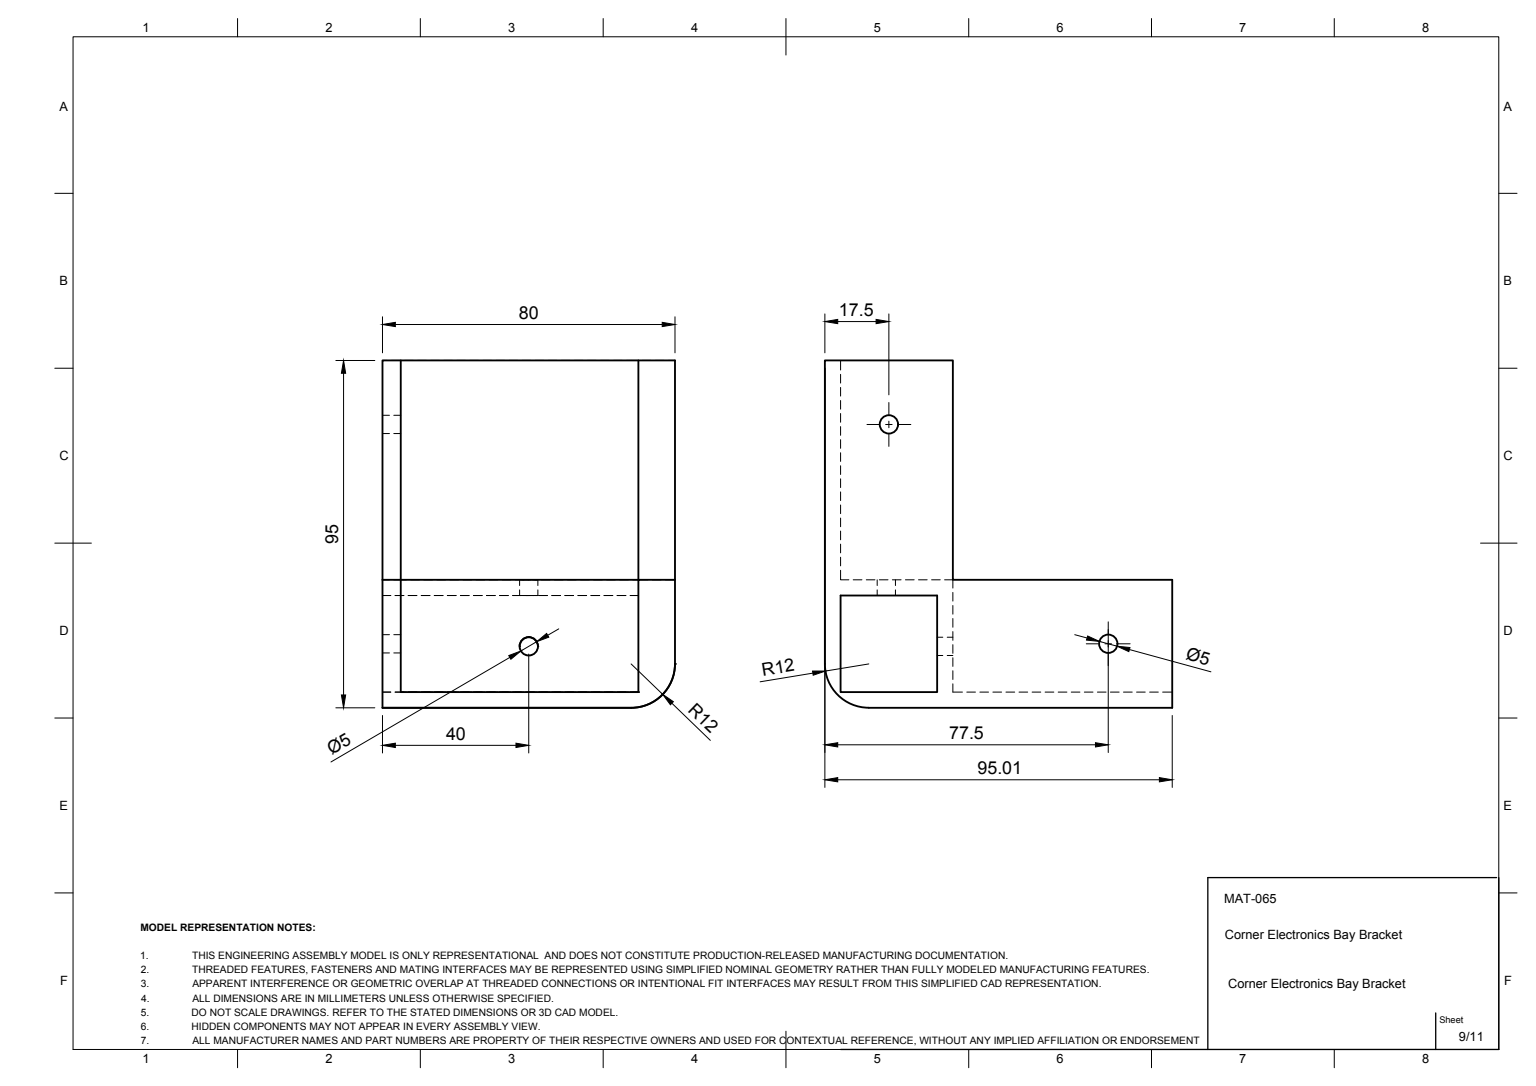
ISO-10303-21;
HEADER;
/* Generated by software containing ST-Developer
 * from STEP Tools, Inc. (www.steptools.com) 
 */

FILE_DESCRIPTION(
/* description */ (
'CAx-IF Rec.Pracs.---Representation and Presentation of Product Manufa
cturing Information (PMI)---4.0---2014-10-13'),
/* implementation_level */ '2;1');

FILE_NAME(
/* name */ 'Corner Electronics Bay Bracket.step',
/* time_stamp */ '2026-11-15T23:28:27-08:00',
/* author */ (''),
/* organization */ (''),
/* preprocessor_version */ 'ST-DEVELOPER v20.2',
/* originating_system */ 'Autodesk Translation Framework v15.17.0.0',
/* authorisation */ '');

FILE_SCHEMA (('AUTOMOTIVE_DESIGN { 1 0 10303 214 3 1 1 }'));
ENDSEC;

DATA;
#10=MECHANICAL_DESIGN_GEOMETRIC_PRESENTATION_REPRESENTATION('',(#196),#7756);
#164=SPHERICAL_SURFACE('',#5002,0.012);
#178=SHAPE_REPRESENTATION_RELATIONSHIP('SRR','None',#7826,#187);
#187=ADVANCED_BREP_SHAPE_REPRESENTATION('',(#205),#7754);
#196=STYLED_ITEM('',(#7874),#205);
#205=MANIFOLD_SOLID_BREP('Body1',#4633);
#239=CYLINDRICAL_SURFACE('',#4970,0.0025);
#240=CYLINDRICAL_SURFACE('',#4977,0.0025);
#241=CYLINDRICAL_SURFACE('',#4988,0.0025);
#242=CYLINDRICAL_SURFACE('',#4989,0.0025);
#243=CYLINDRICAL_SURFACE('',#4996,0.012);
#244=CYLINDRICAL_SURFACE('',#4998,0.012);
#245=CYLINDRICAL_SURFACE('',#5000,0.012);
#328=CIRCLE('',#4959,0.0025);
#329=CIRCLE('',#4963,0.0025);
#330=CIRCLE('',#4967,0.012);
#331=CIRCLE('',#4971,0.0025);
#332=CIRCLE('',#4972,0.0025);
#333=CIRCLE('',#4974,0.0025);
#334=CIRCLE('',#4976,0.012);
#335=CIRCLE('',#4978,0.0025);
#336=CIRCLE('',#4981,0.012);
#337=CIRCLE('',#4983,0.0025);
#338=CIRCLE('',#4987,0.0025);
#339=CIRCLE('',#4997,0.012);
#340=CIRCLE('',#4999,0.012);
#341=CIRCLE('',#5001,0.012);
#420=FACE_BOUND('',#877,.T.);
#421=FACE_BOUND('',#881,.T.);
#422=FACE_BOUND('',#889,.T.);
#423=FACE_BOUND('',#893,.T.);
#424=FACE_BOUND('',#895,.T.);
#425=FACE_BOUND('',#896,.T.);
#426=FACE_BOUND('',#897,.T.);
#427=FACE_BOUND('',#899,.T.);
#428=FACE_BOUND('',#903,.T.);
#601=FACE_OUTER_BOUND('',#876,.T.);
#602=FACE_OUTER_BOUND('',#878,.T.);
#603=FACE_OUTER_BOUND('',#879,.T.);
#604=FACE_OUTER_BOUND('',#880,.T.);
#605=FACE_OUTER_BOUND('',#882,.T.);
#606=FACE_OUTER_BOUND('',#883,.T.);
#607=FACE_OUTER_BOUND('',#884,.T.);
#608=FACE_OUTER_BOUND('',#885,.T.);
#609=FACE_OUTER_BOUND('',#886,.T.);
#610=FACE_OUTER_BOUND('',#887,.T.);
#611=FACE_OUTER_BOUND('',#888,.T.);
#612=FACE_OUTER_BOUND('',#890,.T.);
#613=FACE_OUTER_BOUND('',#891,.T.);
#614=FACE_OUTER_BOUND('',#892,.T.);
#615=FACE_OUTER_BOUND('',#894,.T.);
#616=FACE_OUTER_BOUND('',#898,.T.);
#617=FACE_OUTER_BOUND('',#900,.T.);
#618=FACE_OUTER_BOUND('',#901,.T.);
#619=FACE_OUTER_BOUND('',#902,.T.);
#620=FACE_OUTER_BOUND('',#904,.T.);
#621=FACE_OUTER_BOUND('',#905,.T.);
#622=FACE_OUTER_BOUND('',#906,.T.);
#623=FACE_OUTER_BOUND('',#907,.T.);
#624=FACE_OUTER_BOUND('',#908,.T.);
#625=FACE_OUTER_BOUND('',#909,.T.);
#626=FACE_OUTER_BOUND('',#910,.T.);
#627=FACE_OUTER_BOUND('',#911,.T.);
#628=FACE_OUTER_BOUND('',#912,.T.);
#629=FACE_OUTER_BOUND('',#913,.T.);
#630=FACE_OUTER_BOUND('',#914,.T.);
#631=FACE_OUTER_BOUND('',#915,.T.);
#876=EDGE_LOOP('',(#3789,#3790,#3791,#3792));
#877=EDGE_LOOP('',(#3793));
#878=EDGE_LOOP('',(#3794,#3795,#3796,#3797));
#879=EDGE_LOOP('',(#3798,#3799,#3800,#3801));
#880=EDGE_LOOP('',(#3802,#3803,#3804,#3805));
#881=EDGE_LOOP('',(#3806));
#882=EDGE_LOOP('',(#3807,#3808,#3809,#3810));
#883=EDGE_LOOP('',(#3811,#3812,#3813,#3814));
#884=EDGE_LOOP('',(#3815,#3816,#3817,#3818,#3819,#3820,#3821,#3822,#3823));
#885=EDGE_LOOP('',(#3824,#3825,#3826,#3827));
#886=EDGE_LOOP('',(#3828,#3829,#3830,#3831));
#887=EDGE_LOOP('',(#3832,#3833,#3834,#3835));
#888=EDGE_LOOP('',(#3836,#3837,#3838,#3839));
#889=EDGE_LOOP('',(#3840));
#890=EDGE_LOOP('',(#3841,#3842,#3843,#3844,#3845,#3846,#3847,#3848,#3849));
#891=EDGE_LOOP('',(#3850,#3851,#3852,#3853));
#892=EDGE_LOOP('',(#3854,#3855,#3856,#3857));
#893=EDGE_LOOP('',(#3858));
#894=EDGE_LOOP('',(#3859,#3860,#3861,#3862,#3863,#3864,#3865));
#895=EDGE_LOOP('',(#3866,#3867,#3868,#3869));
#896=EDGE_LOOP('',(#3870));
#897=EDGE_LOOP('',(#3871));
#898=EDGE_LOOP('',(#3872,#3873,#3874,#3875));
#899=EDGE_LOOP('',(#3876));
#900=EDGE_LOOP('',(#3877,#3878,#3879,#3880));
#901=EDGE_LOOP('',(#3881,#3882,#3883,#3884));
#902=EDGE_LOOP('',(#3885,#3886,#3887,#3888));
#903=EDGE_LOOP('',(#3889));
#904=EDGE_LOOP('',(#3890,#3891,#3892,#3893));
#905=EDGE_LOOP('',(#3894,#3895,#3896,#3897));
#906=EDGE_LOOP('',(#3898,#3899,#3900,#3901,#3902,#3903));
#907=EDGE_LOOP('',(#3904,#3905,#3906,#3907));
#908=EDGE_LOOP('',(#3908,#3909,#3910,#3911));
#909=EDGE_LOOP('',(#3912,#3913,#3914,#3915));
#910=EDGE_LOOP('',(#3916,#3917,#3918,#3919));
#911=EDGE_LOOP('',(#3920,#3921,#3922,#3923));
#912=EDGE_LOOP('',(#3924,#3925,#3926,#3927));
#913=EDGE_LOOP('',(#3928,#3929,#3930,#3931));
#914=EDGE_LOOP('',(#3932,#3933,#3934,#3935));
#915=EDGE_LOOP('',(#3936,#3937,#3938));
#1323=LINE('',#7251,#1816);
#1324=LINE('',#7253,#1817);
#1325=LINE('',#7255,#1818);
#1326=LINE('',#7256,#1819);
#1327=LINE('',#7262,#1820);
#1328=LINE('',#7264,#1821);
#1329=LINE('',#7266,#1822);
#1330=LINE('',#7267,#1823);
#1331=LINE('',#7270,#1824);
#1332=LINE('',#7272,#1825);
#1333=LINE('',#7273,#1826);
#1334=LINE('',#7276,#1827);
#1335=LINE('',#7278,#1828);
#1336=LINE('',#7279,#1829);
#1337=LINE('',#7285,#1830);
#1338=LINE('',#7287,#1831);
#1339=LINE('',#7289,#1832);
#1340=LINE('',#7290,#1833);
#1341=LINE('',#7294,#1834);
#1342=LINE('',#7296,#1835);
#1343=LINE('',#7298,#1836);
#1344=LINE('',#7299,#1837);
#1345=LINE('',#7303,#1838);
#1346=LINE('',#7306,#1839);
#1347=LINE('',#7308,#1840);
#1348=LINE('',#7310,#1841);
#1349=LINE('',#7312,#1842);
#1350=LINE('',#7314,#1843);
#1351=LINE('',#7315,#1844);
#1352=LINE('',#7318,#1845);
#1353=LINE('',#7319,#1846);
#1354=LINE('',#7320,#1847);
#1355=LINE('',#7323,#1848);
#1356=LINE('',#7324,#1849);
#1357=LINE('',#7329,#1850);
#1358=LINE('',#7332,#1851);
#1359=LINE('',#7333,#1852);
#1360=LINE('',#7340,#1853);
#1361=LINE('',#7342,#1854);
#1362=LINE('',#7344,#1855);
#1363=LINE('',#7345,#1856);
#1364=LINE('',#7346,#1857);
#1365=LINE('',#7349,#1858);
#1366=LINE('',#7353,#1859);
#1367=LINE('',#7354,#1860);
#1368=LINE('',#7359,#1861);
#1369=LINE('',#7361,#1862);
#1370=LINE('',#7362,#1863);
#1371=LINE('',#7366,#1864);
#1372=LINE('',#7369,#1865);
#1373=LINE('',#7370,#1866);
#1374=LINE('',#7372,#1867);
#1375=LINE('',#7376,#1868);
#1376=LINE('',#7378,#1869);
#1377=LINE('',#7381,#1870);
#1378=LINE('',#7382,#1871);
#1379=LINE('',#7384,#1872);
#1380=LINE('',#7385,#1873);
#1381=LINE('',#7387,#1874);
#1382=LINE('',#7388,#1875);
#1383=LINE('',#7390,#1876);
#1816=VECTOR('',#5911,1.);
#1817=VECTOR('',#5912,1.);
#1818=VECTOR('',#5913,1.);
#1819=VECTOR('',#5914,1.);
#1820=VECTOR('',#5919,1.);
#1821=VECTOR('',#5920,1.);
#1822=VECTOR('',#5921,1.);
#1823=VECTOR('',#5922,1.);
#1824=VECTOR('',#5925,1.);
#1825=VECTOR('',#5926,1.);
#1826=VECTOR('',#5927,1.);
#1827=VECTOR('',#5930,1.);
#1828=VECTOR('',#5931,1.);
#1829=VECTOR('',#5932,1.);
#1830=VECTOR('',#5937,1.);
#1831=VECTOR('',#5938,1.);
#1832=VECTOR('',#5939,1.);
#1833=VECTOR('',#5940,1.);
#1834=VECTOR('',#5943,1.);
#1835=VECTOR('',#5944,1.);
#1836=VECTOR('',#5945,1.);
#1837=VECTOR('',#5946,1.);
#1838=VECTOR('',#5949,1.);
#1839=VECTOR('',#5952,1.);
#1840=VECTOR('',#5953,1.);
#1841=VECTOR('',#5954,1.);
#1842=VECTOR('',#5955,1.);
#1843=VECTOR('',#5956,1.);
#1844=VECTOR('',#5957,1.);
#1845=VECTOR('',#5960,1.);
#1846=VECTOR('',#5961,1.);
#1847=VECTOR('',#5962,1.);
#1848=VECTOR('',#5965,1.);
#1849=VECTOR('',#5966,1.);
#1850=VECTOR('',#5971,0.0025);
#1851=VECTOR('',#5976,1.);
#1852=VECTOR('',#5977,1.);
#1853=VECTOR('',#5984,1.);
#1854=VECTOR('',#5985,1.);
#1855=VECTOR('',#5986,1.);
#1856=VECTOR('',#5987,1.);
#1857=VECTOR('',#5988,1.);
#1858=VECTOR('',#5991,0.0025);
#1859=VECTOR('',#5996,1.);
#1860=VECTOR('',#5997,1.);
#1861=VECTOR('',#6004,1.);
#1862=VECTOR('',#6005,1.);
#1863=VECTOR('',#6006,1.);
#1864=VECTOR('',#6011,1.);
#1865=VECTOR('',#6014,1.);
#1866=VECTOR('',#6015,1.);
#1867=VECTOR('',#6018,1.);
#1868=VECTOR('',#6023,0.0025);
#1869=VECTOR('',#6026,0.0025);
#1870=VECTOR('',#6029,1.);
#1871=VECTOR('',#6030,1.);
#1872=VECTOR('',#6031,1.);
#1873=VECTOR('',#6032,1.);
#1874=VECTOR('',#6035,1.);
#1875=VECTOR('',#6036,1.);
#1876=VECTOR('',#6039,1.);
#2241=VERTEX_POINT('',#7249);
#2242=VERTEX_POINT('',#7250);
#2243=VERTEX_POINT('',#7252);
#2244=VERTEX_POINT('',#7254);
#2245=VERTEX_POINT('',#7257);
#2246=VERTEX_POINT('',#7260);
#2247=VERTEX_POINT('',#7261);
#2248=VERTEX_POINT('',#7263);
#2249=VERTEX_POINT('',#7265);
#2250=VERTEX_POINT('',#7269);
#2251=VERTEX_POINT('',#7271);
#2252=VERTEX_POINT('',#7275);
#2253=VERTEX_POINT('',#7277);
#2254=VERTEX_POINT('',#7280);
#2255=VERTEX_POINT('',#7283);
#2256=VERTEX_POINT('',#7284);
#2257=VERTEX_POINT('',#7286);
#2258=VERTEX_POINT('',#7288);
#2259=VERTEX_POINT('',#7292);
#2260=VERTEX_POINT('',#7293);
#2261=VERTEX_POINT('',#7295);
#2262=VERTEX_POINT('',#7297);
#2263=VERTEX_POINT('',#7301);
#2264=VERTEX_POINT('',#7302);
#2265=VERTEX_POINT('',#7305);
#2266=VERTEX_POINT('',#7307);
#2267=VERTEX_POINT('',#7309);
#2268=VERTEX_POINT('',#7311);
#2269=VERTEX_POINT('',#7313);
#2270=VERTEX_POINT('',#7317);
#2271=VERTEX_POINT('',#7322);
#2272=VERTEX_POINT('',#7326);
#2273=VERTEX_POINT('',#7328);
#2274=VERTEX_POINT('',#7334);
#2275=VERTEX_POINT('',#7337);
#2276=VERTEX_POINT('',#7339);
#2277=VERTEX_POINT('',#7341);
#2278=VERTEX_POINT('',#7343);
#2279=VERTEX_POINT('',#7348);
#2280=VERTEX_POINT('',#7352);
#2281=VERTEX_POINT('',#7358);
#2282=VERTEX_POINT('',#7360);
#2283=VERTEX_POINT('',#7363);
#2284=VERTEX_POINT('',#7368);
#2285=VERTEX_POINT('',#7373);
#2286=VERTEX_POINT('',#7380);
#2287=VERTEX_POINT('',#7383);
#2778=EDGE_CURVE('',#2241,#2242,#1323,.T.);
#2779=EDGE_CURVE('',#2241,#2243,#1324,.T.);
#2780=EDGE_CURVE('',#2243,#2244,#1325,.T.);
#2781=EDGE_CURVE('',#2244,#2242,#1326,.T.);
#2782=EDGE_CURVE('',#2245,#2245,#328,.T.);
#2783=EDGE_CURVE('',#2246,#2247,#1327,.T.);
#2784=EDGE_CURVE('',#2248,#2246,#1328,.T.);
#2785=EDGE_CURVE('',#2248,#2249,#1329,.T.);
#2786=EDGE_CURVE('',#2249,#2247,#1330,.T.);
#2787=EDGE_CURVE('',#2246,#2250,#1331,.T.);
#2788=EDGE_CURVE('',#2251,#2250,#1332,.T.);
#2789=EDGE_CURVE('',#2248,#2251,#1333,.T.);
#2790=EDGE_CURVE('',#2250,#2252,#1334,.T.);
#2791=EDGE_CURVE('',#2253,#2252,#1335,.T.);
#2792=EDGE_CURVE('',#2251,#2253,#1336,.T.);
#2793=EDGE_CURVE('',#2254,#2254,#329,.T.);
#2794=EDGE_CURVE('',#2255,#2256,#1337,.F.);
#2795=EDGE_CURVE('',#2256,#2257,#1338,.T.);
#2796=EDGE_CURVE('',#2257,#2258,#1339,.T.);
#2797=EDGE_CURVE('',#2255,#2258,#1340,.T.);
#2798=EDGE_CURVE('',#2259,#2260,#1341,.T.);
#2799=EDGE_CURVE('',#2259,#2261,#1342,.T.);
#2800=EDGE_CURVE('',#2261,#2262,#1343,.T.);
#2801=EDGE_CURVE('',#2260,#2262,#1344,.T.);
#2802=EDGE_CURVE('',#2263,#2264,#1345,.T.);
#2803=EDGE_CURVE('',#2263,#2259,#330,.F.);
#2804=EDGE_CURVE('',#2260,#2265,#1346,.T.);
#2805=EDGE_CURVE('',#2266,#2265,#1347,.T.);
#2806=EDGE_CURVE('',#2267,#2266,#1348,.T.);
#2807=EDGE_CURVE('',#2268,#2267,#1349,.T.);
#2808=EDGE_CURVE('',#2268,#2269,#1350,.T.);
#2809=EDGE_CURVE('',#2264,#2269,#1351,.T.);
#2810=EDGE_CURVE('',#2265,#2270,#1352,.T.);
#2811=EDGE_CURVE('',#2243,#2270,#1353,.T.);
#2812=EDGE_CURVE('',#2266,#2243,#1354,.T.);
#2813=EDGE_CURVE('',#2270,#2271,#1355,.T.);
#2814=EDGE_CURVE('',#2244,#2271,#1356,.T.);
#2815=EDGE_CURVE('',#2272,#2272,#331,.T.);
#2816=EDGE_CURVE('',#2272,#2273,#1357,.T.);
#2817=EDGE_CURVE('',#2273,#2273,#332,.T.);
#2818=EDGE_CURVE('',#2247,#2252,#1358,.T.);
#2819=EDGE_CURVE('',#2249,#2253,#1359,.T.);
#2820=EDGE_CURVE('',#2274,#2274,#333,.T.);
#2821=EDGE_CURVE('',#2257,#2275,#334,.F.);
#2822=EDGE_CURVE('',#2275,#2276,#1360,.T.);
#2823=EDGE_CURVE('',#2276,#2277,#1361,.T.);
#2824=EDGE_CURVE('',#2278,#2277,#1362,.T.);
#2825=EDGE_CURVE('',#2278,#2242,#1363,.T.);
#2826=EDGE_CURVE('',#2271,#2258,#1364,.T.);
#2827=EDGE_CURVE('',#2245,#2279,#1365,.T.);
#2828=EDGE_CURVE('',#2279,#2279,#335,.T.);
#2829=EDGE_CURVE('',#2267,#2280,#1366,.T.);
#2830=EDGE_CURVE('',#2280,#2243,#1367,.T.);
#2831=EDGE_CURVE('',#2262,#2255,#336,.F.);
#2832=EDGE_CURVE('',#2281,#2241,#1368,.T.);
#2833=EDGE_CURVE('',#2281,#2282,#1369,.T.);
#2834=EDGE_CURVE('',#2282,#2243,#1370,.T.);
#2835=EDGE_CURVE('',#2283,#2283,#337,.T.);
#2836=EDGE_CURVE('',#2281,#2278,#1371,.T.);
#2837=EDGE_CURVE('',#2284,#2280,#1372,.T.);
#2838=EDGE_CURVE('',#2268,#2284,#1373,.T.);
#2839=EDGE_CURVE('',#2284,#2282,#1374,.T.);
#2840=EDGE_CURVE('',#2285,#2285,#338,.T.);
#2841=EDGE_CURVE('',#2254,#2283,#1375,.T.);
#2842=EDGE_CURVE('',#2274,#2285,#1376,.T.);
#2843=EDGE_CURVE('',#2275,#2286,#1377,.F.);
#2844=EDGE_CURVE('',#2286,#2263,#1378,.F.);
#2845=EDGE_CURVE('',#2264,#2287,#1379,.T.);
#2846=EDGE_CURVE('',#2276,#2287,#1380,.T.);
#2847=EDGE_CURVE('',#2277,#2282,#1381,.T.);
#2848=EDGE_CURVE('',#2287,#2282,#1382,.T.);
#2849=EDGE_CURVE('',#2269,#2282,#1383,.T.);
#2850=EDGE_CURVE('',#2261,#2256,#339,.T.);
#2851=EDGE_CURVE('',#2286,#2261,#340,.F.);
#2852=EDGE_CURVE('',#2286,#2256,#341,.T.);
#3789=ORIENTED_EDGE('',*,*,#2778,.F.);
#3790=ORIENTED_EDGE('',*,*,#2779,.T.);
#3791=ORIENTED_EDGE('',*,*,#2780,.T.);
#3792=ORIENTED_EDGE('',*,*,#2781,.T.);
#3793=ORIENTED_EDGE('',*,*,#2782,.T.);
#3794=ORIENTED_EDGE('',*,*,#2783,.F.);
#3795=ORIENTED_EDGE('',*,*,#2784,.F.);
#3796=ORIENTED_EDGE('',*,*,#2785,.T.);
#3797=ORIENTED_EDGE('',*,*,#2786,.T.);
#3798=ORIENTED_EDGE('',*,*,#2787,.T.);
#3799=ORIENTED_EDGE('',*,*,#2788,.F.);
#3800=ORIENTED_EDGE('',*,*,#2789,.F.);
#3801=ORIENTED_EDGE('',*,*,#2784,.T.);
#3802=ORIENTED_EDGE('',*,*,#2790,.T.);
#3803=ORIENTED_EDGE('',*,*,#2791,.F.);
#3804=ORIENTED_EDGE('',*,*,#2792,.F.);
#3805=ORIENTED_EDGE('',*,*,#2788,.T.);
#3806=ORIENTED_EDGE('',*,*,#2793,.T.);
#3807=ORIENTED_EDGE('',*,*,#2794,.T.);
#3808=ORIENTED_EDGE('',*,*,#2795,.T.);
#3809=ORIENTED_EDGE('',*,*,#2796,.T.);
#3810=ORIENTED_EDGE('',*,*,#2797,.F.);
#3811=ORIENTED_EDGE('',*,*,#2798,.F.);
#3812=ORIENTED_EDGE('',*,*,#2799,.T.);
#3813=ORIENTED_EDGE('',*,*,#2800,.T.);
#3814=ORIENTED_EDGE('',*,*,#2801,.F.);
#3815=ORIENTED_EDGE('',*,*,#2802,.F.);
#3816=ORIENTED_EDGE('',*,*,#2803,.T.);
#3817=ORIENTED_EDGE('',*,*,#2798,.T.);
#3818=ORIENTED_EDGE('',*,*,#2804,.T.);
#3819=ORIENTED_EDGE('',*,*,#2805,.F.);
#3820=ORIENTED_EDGE('',*,*,#2806,.F.);
#3821=ORIENTED_EDGE('',*,*,#2807,.F.);
#3822=ORIENTED_EDGE('',*,*,#2808,.T.);
#3823=ORIENTED_EDGE('',*,*,#2809,.F.);
#3824=ORIENTED_EDGE('',*,*,#2810,.T.);
#3825=ORIENTED_EDGE('',*,*,#2811,.F.);
#3826=ORIENTED_EDGE('',*,*,#2812,.F.);
#3827=ORIENTED_EDGE('',*,*,#2805,.T.);
#3828=ORIENTED_EDGE('',*,*,#2813,.T.);
#3829=ORIENTED_EDGE('',*,*,#2814,.F.);
#3830=ORIENTED_EDGE('',*,*,#2780,.F.);
#3831=ORIENTED_EDGE('',*,*,#2811,.T.);
#3832=ORIENTED_EDGE('',*,*,#2815,.F.);
#3833=ORIENTED_EDGE('',*,*,#2816,.T.);
#3834=ORIENTED_EDGE('',*,*,#2817,.T.);
#3835=ORIENTED_EDGE('',*,*,#2816,.F.);
#3836=ORIENTED_EDGE('',*,*,#2818,.F.);
#3837=ORIENTED_EDGE('',*,*,#2786,.F.);
#3838=ORIENTED_EDGE('',*,*,#2819,.T.);
#3839=ORIENTED_EDGE('',*,*,#2791,.T.);
#3840=ORIENTED_EDGE('',*,*,#2820,.F.);
#3841=ORIENTED_EDGE('',*,*,#2796,.F.);
#3842=ORIENTED_EDGE('',*,*,#2821,.T.);
#3843=ORIENTED_EDGE('',*,*,#2822,.T.);
#3844=ORIENTED_EDGE('',*,*,#2823,.T.);
#3845=ORIENTED_EDGE('',*,*,#2824,.F.);
#3846=ORIENTED_EDGE('',*,*,#2825,.T.);
#3847=ORIENTED_EDGE('',*,*,#2781,.F.);
#3848=ORIENTED_EDGE('',*,*,#2814,.T.);
#3849=ORIENTED_EDGE('',*,*,#2826,.T.);
#3850=ORIENTED_EDGE('',*,*,#2782,.F.);
#3851=ORIENTED_EDGE('',*,*,#2827,.T.);
#3852=ORIENTED_EDGE('',*,*,#2828,.T.);
#3853=ORIENTED_EDGE('',*,*,#2827,.F.);
#3854=ORIENTED_EDGE('',*,*,#2829,.F.);
#3855=ORIENTED_EDGE('',*,*,#2806,.T.);
#3856=ORIENTED_EDGE('',*,*,#2812,.T.);
#3857=ORIENTED_EDGE('',*,*,#2830,.F.);
#3858=ORIENTED_EDGE('',*,*,#2815,.T.);
#3859=ORIENTED_EDGE('',*,*,#2801,.T.);
#3860=ORIENTED_EDGE('',*,*,#2831,.T.);
#3861=ORIENTED_EDGE('',*,*,#2797,.T.);
#3862=ORIENTED_EDGE('',*,*,#2826,.F.);
#3863=ORIENTED_EDGE('',*,*,#2813,.F.);
#3864=ORIENTED_EDGE('',*,*,#2810,.F.);
#3865=ORIENTED_EDGE('',*,*,#2804,.F.);
#3866=ORIENTED_EDGE('',*,*,#2783,.T.);
#3867=ORIENTED_EDGE('',*,*,#2818,.T.);
#3868=ORIENTED_EDGE('',*,*,#2790,.F.);
#3869=ORIENTED_EDGE('',*,*,#2787,.F.);
#3870=ORIENTED_EDGE('',*,*,#2817,.F.);
#3871=ORIENTED_EDGE('',*,*,#2828,.F.);
#3872=ORIENTED_EDGE('',*,*,#2779,.F.);
#3873=ORIENTED_EDGE('',*,*,#2832,.F.);
#3874=ORIENTED_EDGE('',*,*,#2833,.T.);
#3875=ORIENTED_EDGE('',*,*,#2834,.T.);
#3876=ORIENTED_EDGE('',*,*,#2835,.F.);
#3877=ORIENTED_EDGE('',*,*,#2778,.T.);
#3878=ORIENTED_EDGE('',*,*,#2825,.F.);
#3879=ORIENTED_EDGE('',*,*,#2836,.F.);
#3880=ORIENTED_EDGE('',*,*,#2832,.T.);
#3881=ORIENTED_EDGE('',*,*,#2829,.T.);
#3882=ORIENTED_EDGE('',*,*,#2837,.F.);
#3883=ORIENTED_EDGE('',*,*,#2838,.F.);
#3884=ORIENTED_EDGE('',*,*,#2807,.T.);
#3885=ORIENTED_EDGE('',*,*,#2830,.T.);
#3886=ORIENTED_EDGE('',*,*,#2834,.F.);
#3887=ORIENTED_EDGE('',*,*,#2839,.F.);
#3888=ORIENTED_EDGE('',*,*,#2837,.T.);
#3889=ORIENTED_EDGE('',*,*,#2840,.F.);
#3890=ORIENTED_EDGE('',*,*,#2793,.F.);
#3891=ORIENTED_EDGE('',*,*,#2841,.T.);
#3892=ORIENTED_EDGE('',*,*,#2835,.T.);
#3893=ORIENTED_EDGE('',*,*,#2841,.F.);
#3894=ORIENTED_EDGE('',*,*,#2820,.T.);
#3895=ORIENTED_EDGE('',*,*,#2842,.T.);
#3896=ORIENTED_EDGE('',*,*,#2840,.T.);
#3897=ORIENTED_EDGE('',*,*,#2842,.F.);
#3898=ORIENTED_EDGE('',*,*,#2822,.F.);
#3899=ORIENTED_EDGE('',*,*,#2843,.T.);
#3900=ORIENTED_EDGE('',*,*,#2844,.T.);
#3901=ORIENTED_EDGE('',*,*,#2802,.T.);
#3902=ORIENTED_EDGE('',*,*,#2845,.T.);
#3903=ORIENTED_EDGE('',*,*,#2846,.F.);
#3904=ORIENTED_EDGE('',*,*,#2847,.F.);
#3905=ORIENTED_EDGE('',*,*,#2823,.F.);
#3906=ORIENTED_EDGE('',*,*,#2846,.T.);
#3907=ORIENTED_EDGE('',*,*,#2848,.T.);
#3908=ORIENTED_EDGE('',*,*,#2849,.T.);
#3909=ORIENTED_EDGE('',*,*,#2848,.F.);
#3910=ORIENTED_EDGE('',*,*,#2845,.F.);
#3911=ORIENTED_EDGE('',*,*,#2809,.T.);
#3912=ORIENTED_EDGE('',*,*,#2808,.F.);
#3913=ORIENTED_EDGE('',*,*,#2838,.T.);
#3914=ORIENTED_EDGE('',*,*,#2839,.T.);
#3915=ORIENTED_EDGE('',*,*,#2849,.F.);
#3916=ORIENTED_EDGE('',*,*,#2833,.F.);
#3917=ORIENTED_EDGE('',*,*,#2836,.T.);
#3918=ORIENTED_EDGE('',*,*,#2824,.T.);
#3919=ORIENTED_EDGE('',*,*,#2847,.T.);
#3920=ORIENTED_EDGE('',*,*,#2785,.F.);
#3921=ORIENTED_EDGE('',*,*,#2789,.T.);
#3922=ORIENTED_EDGE('',*,*,#2792,.T.);
#3923=ORIENTED_EDGE('',*,*,#2819,.F.);
#3924=ORIENTED_EDGE('',*,*,#2800,.F.);
#3925=ORIENTED_EDGE('',*,*,#2850,.T.);
#3926=ORIENTED_EDGE('',*,*,#2794,.F.);
#3927=ORIENTED_EDGE('',*,*,#2831,.F.);
#3928=ORIENTED_EDGE('',*,*,#2844,.F.);
#3929=ORIENTED_EDGE('',*,*,#2851,.T.);
#3930=ORIENTED_EDGE('',*,*,#2799,.F.);
#3931=ORIENTED_EDGE('',*,*,#2803,.F.);
#3932=ORIENTED_EDGE('',*,*,#2821,.F.);
#3933=ORIENTED_EDGE('',*,*,#2795,.F.);
#3934=ORIENTED_EDGE('',*,*,#2852,.F.);
#3935=ORIENTED_EDGE('',*,*,#2843,.F.);
#3936=ORIENTED_EDGE('',*,*,#2852,.T.);
#3937=ORIENTED_EDGE('',*,*,#2850,.F.);
#3938=ORIENTED_EDGE('',*,*,#2851,.F.);
#4335=PLANE('',#4958);
#4336=PLANE('',#4960);
#4337=PLANE('',#4961);
#4338=PLANE('',#4962);
#4339=PLANE('',#4964);
#4340=PLANE('',#4965);
#4341=PLANE('',#4966);
#4342=PLANE('',#4968);
#4343=PLANE('',#4969);
#4344=PLANE('',#4973);
#4345=PLANE('',#4975);
#4346=PLANE('',#4979);
#4347=PLANE('',#4980);
#4348=PLANE('',#4982);
#4349=PLANE('',#4984);
#4350=PLANE('',#4985);
#4351=PLANE('',#4986);
#4352=PLANE('',#4990);
#4353=PLANE('',#4991);
#4354=PLANE('',#4992);
#4355=PLANE('',#4993);
#4356=PLANE('',#4994);
#4357=PLANE('',#4995);
#4542=ADVANCED_FACE('',(#601,#420),#4335,.T.);
#4543=ADVANCED_FACE('',(#602),#4336,.T.);
#4544=ADVANCED_FACE('',(#603),#4337,.F.);
#4545=ADVANCED_FACE('',(#604,#421),#4338,.F.);
#4546=ADVANCED_FACE('',(#605),#4339,.T.);
#4547=ADVANCED_FACE('',(#606),#4340,.T.);
#4548=ADVANCED_FACE('',(#607),#4341,.F.);
#4549=ADVANCED_FACE('',(#608),#4342,.F.);
#4550=ADVANCED_FACE('',(#609),#4343,.F.);
#4551=ADVANCED_FACE('',(#610),#239,.F.);
#4552=ADVANCED_FACE('',(#611,#422),#4344,.T.);
#4553=ADVANCED_FACE('',(#612),#4345,.F.);
#4554=ADVANCED_FACE('',(#613),#240,.F.);
#4555=ADVANCED_FACE('',(#614,#423),#4346,.T.);
#4556=ADVANCED_FACE('',(#615,#424,#425,#426),#4347,.F.);
#4557=ADVANCED_FACE('',(#616,#427),#4348,.T.);
#4558=ADVANCED_FACE('',(#617),#4349,.F.);
#4559=ADVANCED_FACE('',(#618),#4350,.F.);
#4560=ADVANCED_FACE('',(#619,#428),#4351,.F.);
#4561=ADVANCED_FACE('',(#620),#241,.F.);
#4562=ADVANCED_FACE('',(#621),#242,.F.);
#4563=ADVANCED_FACE('',(#622),#4352,.T.);
#4564=ADVANCED_FACE('',(#623),#4353,.T.);
#4565=ADVANCED_FACE('',(#624),#4354,.F.);
#4566=ADVANCED_FACE('',(#625),#4355,.F.);
#4567=ADVANCED_FACE('',(#626),#4356,.F.);
#4568=ADVANCED_FACE('',(#627),#4357,.F.);
#4569=ADVANCED_FACE('',(#628),#243,.T.);
#4570=ADVANCED_FACE('',(#629),#244,.T.);
#4571=ADVANCED_FACE('',(#630),#245,.T.);
#4572=ADVANCED_FACE('',(#631),#164,.T.);
#4633=CLOSED_SHELL('',(#4542,#4543,#4544,#4545,#4546,#4547,#4548,#4549,
#4550,#4551,#4552,#4553,#4554,#4555,#4556,#4557,#4558,#4559,#4560,#4561,
#4562,#4563,#4564,#4565,#4566,#4567,#4568,#4569,#4570,#4571,#4572));
#4957=AXIS2_PLACEMENT_3D('',#7247,#5907,#5908);
#4958=AXIS2_PLACEMENT_3D('',#7248,#5909,#5910);
#4959=AXIS2_PLACEMENT_3D('',#7258,#5915,#5916);
#4960=AXIS2_PLACEMENT_3D('',#7259,#5917,#5918);
#4961=AXIS2_PLACEMENT_3D('',#7268,#5923,#5924);
#4962=AXIS2_PLACEMENT_3D('',#7274,#5928,#5929);
#4963=AXIS2_PLACEMENT_3D('',#7281,#5933,#5934);
#4964=AXIS2_PLACEMENT_3D('',#7282,#5935,#5936);
#4965=AXIS2_PLACEMENT_3D('',#7291,#5941,#5942);
#4966=AXIS2_PLACEMENT_3D('',#7300,#5947,#5948);
#4967=AXIS2_PLACEMENT_3D('',#7304,#5950,#5951);
#4968=AXIS2_PLACEMENT_3D('',#7316,#5958,#5959);
#4969=AXIS2_PLACEMENT_3D('',#7321,#5963,#5964);
#4970=AXIS2_PLACEMENT_3D('',#7325,#5967,#5968);
#4971=AXIS2_PLACEMENT_3D('',#7327,#5969,#5970);
#4972=AXIS2_PLACEMENT_3D('',#7330,#5972,#5973);
#4973=AXIS2_PLACEMENT_3D('',#7331,#5974,#5975);
#4974=AXIS2_PLACEMENT_3D('',#7335,#5978,#5979);
#4975=AXIS2_PLACEMENT_3D('',#7336,#5980,#5981);
#4976=AXIS2_PLACEMENT_3D('',#7338,#5982,#5983);
#4977=AXIS2_PLACEMENT_3D('',#7347,#5989,#5990);
#4978=AXIS2_PLACEMENT_3D('',#7350,#5992,#5993);
#4979=AXIS2_PLACEMENT_3D('',#7351,#5994,#5995);
#4980=AXIS2_PLACEMENT_3D('',#7355,#5998,#5999);
#4981=AXIS2_PLACEMENT_3D('',#7356,#6000,#6001);
#4982=AXIS2_PLACEMENT_3D('',#7357,#6002,#6003);
#4983=AXIS2_PLACEMENT_3D('',#7364,#6007,#6008);
#4984=AXIS2_PLACEMENT_3D('',#7365,#6009,#6010);
#4985=AXIS2_PLACEMENT_3D('',#7367,#6012,#6013);
#4986=AXIS2_PLACEMENT_3D('',#7371,#6016,#6017);
#4987=AXIS2_PLACEMENT_3D('',#7374,#6019,#6020);
#4988=AXIS2_PLACEMENT_3D('',#7375,#6021,#6022);
#4989=AXIS2_PLACEMENT_3D('',#7377,#6024,#6025);
#4990=AXIS2_PLACEMENT_3D('',#7379,#6027,#6028);
#4991=AXIS2_PLACEMENT_3D('',#7386,#6033,#6034);
#4992=AXIS2_PLACEMENT_3D('',#7389,#6037,#6038);
#4993=AXIS2_PLACEMENT_3D('',#7391,#6040,#6041);
#4994=AXIS2_PLACEMENT_3D('',#7392,#6042,#6043);
#4995=AXIS2_PLACEMENT_3D('',#7393,#6044,#6045);
#4996=AXIS2_PLACEMENT_3D('',#7394,#6046,#6047);
#4997=AXIS2_PLACEMENT_3D('',#7395,#6048,#6049);
#4998=AXIS2_PLACEMENT_3D('',#7396,#6050,#6051);
#4999=AXIS2_PLACEMENT_3D('',#7397,#6052,#6053);
#5000=AXIS2_PLACEMENT_3D('',#7398,#6054,#6055);
#5001=AXIS2_PLACEMENT_3D('',#7399,#6056,#6057);
#5002=AXIS2_PLACEMENT_3D('',#7400,#6058,#6059);
#5907=DIRECTION('axis',(0.,0.,1.));
#5908=DIRECTION('refdir',(1.,0.,0.));
#5909=DIRECTION('center_axis',(0.,0.,-1.));
#5910=DIRECTION('ref_axis',(1.,0.,0.));
#5911=DIRECTION('',(1.,-4.62592926927149E-16,0.));
#5912=DIRECTION('',(0.,1.,0.));
#5913=DIRECTION('',(1.,0.,0.));
#5914=DIRECTION('',(0.,-1.,0.));
#5915=DIRECTION('center_axis',(0.,0.,1.));
#5916=DIRECTION('ref_axis',(1.,0.,0.));
#5917=DIRECTION('center_axis',(1.,-6.57092225748791E-17,0.));
#5918=DIRECTION('ref_axis',(6.57092225748791E-17,1.,0.));
#5919=DIRECTION('',(6.57092225748791E-17,1.,0.));
#5920=DIRECTION('',(0.,0.,1.));
#5921=DIRECTION('',(6.57092225748791E-17,1.,0.));
#5922=DIRECTION('',(0.,0.,1.));
#5923=DIRECTION('center_axis',(0.,-1.,0.));
#5924=DIRECTION('ref_axis',(0.,0.,-1.));
#5925=DIRECTION('',(1.,0.,0.));
#5926=DIRECTION('',(0.,0.,1.));
#5927=DIRECTION('',(1.,0.,0.));
#5928=DIRECTION('center_axis',(1.,0.,0.));
#5929=DIRECTION('ref_axis',(0.,0.,-1.));
#5930=DIRECTION('',(0.,1.,0.));
#5931=DIRECTION('',(0.,0.,1.));
#5932=DIRECTION('',(0.,1.,0.));
#5933=DIRECTION('center_axis',(1.,0.,0.));
#5934=DIRECTION('ref_axis',(0.,0.,-1.));
#5935=DIRECTION('center_axis',(0.,-1.,0.));
#5936=DIRECTION('ref_axis',(0.,0.,-1.));
#5937=DIRECTION('',(0.,0.,1.));
#5938=DIRECTION('',(1.,0.,0.));
#5939=DIRECTION('',(0.,0.,1.));
#5940=DIRECTION('',(1.,0.,0.));
#5941=DIRECTION('center_axis',(-1.,0.,0.));
#5942=DIRECTION('ref_axis',(0.,0.,1.));
#5943=DIRECTION('',(0.,0.,1.));
#5944=DIRECTION('',(0.,-1.,0.));
#5945=DIRECTION('',(0.,0.,1.));
#5946=DIRECTION('',(0.,-1.,0.));
#5947=DIRECTION('center_axis',(0.,-1.,0.));
#5948=DIRECTION('ref_axis',(0.,0.,-1.));
#5949=DIRECTION('',(1.,0.,0.));
#5950=DIRECTION('center_axis',(0.,-1.,0.));
#5951=DIRECTION('ref_axis',(0.,0.,-1.));
#5952=DIRECTION('',(1.,0.,0.));
#5953=DIRECTION('',(0.,0.,1.));
#5954=DIRECTION('',(1.,0.,0.));
#5955=DIRECTION('',(0.,0.,1.));
#5956=DIRECTION('',(1.,0.,0.));
#5957=DIRECTION('',(0.,0.,1.));
#5958=DIRECTION('center_axis',(-1.,0.,0.));
#5959=DIRECTION('ref_axis',(0.,0.,1.));
#5960=DIRECTION('',(0.,-1.,0.));
#5961=DIRECTION('',(0.,0.,1.));
#5962=DIRECTION('',(0.,-1.,0.));
#5963=DIRECTION('center_axis',(0.,-1.,0.));
#5964=DIRECTION('ref_axis',(0.,0.,-1.));
#5965=DIRECTION('',(1.,0.,0.));
#5966=DIRECTION('',(0.,0.,1.));
#5967=DIRECTION('center_axis',(0.,0.,1.));
#5968=DIRECTION('ref_axis',(1.,0.,0.));
#5969=DIRECTION('center_axis',(0.,0.,1.));
#5970=DIRECTION('ref_axis',(1.,0.,0.));
#5971=DIRECTION('',(0.,0.,1.));
#5972=DIRECTION('center_axis',(0.,0.,1.));
#5973=DIRECTION('ref_axis',(1.,0.,0.));
#5974=DIRECTION('center_axis',(0.,-1.,0.));
#5975=DIRECTION('ref_axis',(0.,0.,-1.));
#5976=DIRECTION('',(1.,0.,0.));
#5977=DIRECTION('',(1.,0.,0.));
#5978=DIRECTION('center_axis',(0.,-1.,0.));
#5979=DIRECTION('ref_axis',(0.,0.,-1.));
#5980=DIRECTION('center_axis',(-1.,0.,0.));
#5981=DIRECTION('ref_axis',(0.,0.,1.));
#5982=DIRECTION('center_axis',(-1.,0.,0.));
#5983=DIRECTION('ref_axis',(0.,0.,1.));
#5984=DIRECTION('',(0.,1.,0.));
#5985=DIRECTION('',(0.,0.,1.));
#5986=DIRECTION('',(0.,1.,0.));
#5987=DIRECTION('',(0.,0.,1.));
#5988=DIRECTION('',(0.,-1.,0.));
#5989=DIRECTION('center_axis',(0.,0.,1.));
#5990=DIRECTION('ref_axis',(1.,0.,0.));
#5991=DIRECTION('',(0.,0.,1.));
#5992=DIRECTION('center_axis',(0.,0.,1.));
#5993=DIRECTION('ref_axis',(1.,0.,0.));
#5994=DIRECTION('center_axis',(0.,0.,-1.));
#5995=DIRECTION('ref_axis',(1.,0.,0.));
#5996=DIRECTION('',(0.,-1.,0.));
#5997=DIRECTION('',(1.,0.,0.));
#5998=DIRECTION('center_axis',(0.,0.,-1.));
#5999=DIRECTION('ref_axis',(1.,0.,0.));
#6000=DIRECTION('center_axis',(0.,0.,-1.));
#6001=DIRECTION('ref_axis',(-1.,0.,0.));
#6002=DIRECTION('center_axis',(1.,0.,0.));
#6003=DIRECTION('ref_axis',(0.,0.,-1.));
#6004=DIRECTION('',(0.,0.,1.));
#6005=DIRECTION('',(0.,1.,0.));
#6006=DIRECTION('',(0.,0.,1.));
#6007=DIRECTION('center_axis',(1.,0.,0.));
#6008=DIRECTION('ref_axis',(0.,0.,-1.));
#6009=DIRECTION('center_axis',(-4.62592926927149E-16,-1.,0.));
#6010=DIRECTION('ref_axis',(1.,-4.62592926927149E-16,0.));
#6011=DIRECTION('',(1.,-4.62592926927149E-16,0.));
#6012=DIRECTION('center_axis',(-1.,0.,0.));
#6013=DIRECTION('ref_axis',(0.,0.,1.));
#6014=DIRECTION('',(0.,0.,1.));
#6015=DIRECTION('',(0.,-1.,0.));
#6016=DIRECTION('center_axis',(0.,-1.,0.));
#6017=DIRECTION('ref_axis',(0.,0.,-1.));
#6018=DIRECTION('',(1.,0.,0.));
#6019=DIRECTION('center_axis',(0.,1.,0.));
#6020=DIRECTION('ref_axis',(0.,0.,1.));
#6021=DIRECTION('center_axis',(1.,0.,0.));
#6022=DIRECTION('ref_axis',(0.,0.,-1.));
#6023=DIRECTION('',(1.,0.,0.));
#6024=DIRECTION('center_axis',(0.,1.,0.));
#6025=DIRECTION('ref_axis',(0.,0.,1.));
#6026=DIRECTION('',(0.,1.,0.));
#6027=DIRECTION('center_axis',(0.,0.,-1.));
#6028=DIRECTION('ref_axis',(1.,0.,0.));
#6029=DIRECTION('',(1.,0.,0.));
#6030=DIRECTION('',(0.,-1.,0.));
#6031=DIRECTION('',(0.,-1.,0.));
#6032=DIRECTION('',(-1.,0.,0.));
#6033=DIRECTION('center_axis',(0.,1.,0.));
#6034=DIRECTION('ref_axis',(0.,0.,1.));
#6035=DIRECTION('',(-1.,0.,0.));
#6036=DIRECTION('',(0.,0.,1.));
#6037=DIRECTION('center_axis',(-1.,0.,0.));
#6038=DIRECTION('ref_axis',(0.,0.,1.));
#6039=DIRECTION('',(0.,-1.,0.));
#6040=DIRECTION('center_axis',(0.,0.,-1.));
#6041=DIRECTION('ref_axis',(1.,0.,0.));
#6042=DIRECTION('center_axis',(0.,0.,-1.));
#6043=DIRECTION('ref_axis',(1.,0.,0.));
#6044=DIRECTION('center_axis',(0.,0.,-1.));
#6045=DIRECTION('ref_axis',(1.,0.,0.));
#6046=DIRECTION('center_axis',(0.,0.,1.));
#6047=DIRECTION('ref_axis',(1.,0.,0.));
#6048=DIRECTION('center_axis',(0.,0.,1.));
#6049=DIRECTION('ref_axis',(1.,0.,0.));
#6050=DIRECTION('center_axis',(0.,-1.,0.));
#6051=DIRECTION('ref_axis',(0.,0.,-1.));
#6052=DIRECTION('center_axis',(0.,-1.,0.));
#6053=DIRECTION('ref_axis',(0.,0.,-1.));
#6054=DIRECTION('center_axis',(1.,0.,0.));
#6055=DIRECTION('ref_axis',(0.,0.,-1.));
#6056=DIRECTION('center_axis',(-1.,0.,0.));
#6057=DIRECTION('ref_axis',(0.,0.,1.));
#6058=DIRECTION('center_axis',(0.,0.,1.));
#6059=DIRECTION('ref_axis',(1.,0.,0.));
#7247=CARTESIAN_POINT('',(0.,0.,0.));
#7248=CARTESIAN_POINT('Origin',(0.0475,-0.015275768481829,-0.005));
#7249=CARTESIAN_POINT('',(0.035,-0.058475768481829,-0.005));
#7250=CARTESIAN_POINT('',(0.095,-0.058475768481829,-0.005));
#7251=CARTESIAN_POINT('',(0.065,-0.058475768481829,-0.005));
#7252=CARTESIAN_POINT('',(0.035,-0.027775768481829,-0.005));
#7253=CARTESIAN_POINT('',(0.035,-0.043125768481829,-0.005));
#7254=CARTESIAN_POINT('',(0.095,-0.027775768481829,-0.005));
#7255=CARTESIAN_POINT('',(0.065,-0.027775768481829,-0.005));
#7256=CARTESIAN_POINT('',(0.095,-0.045275768481829,-0.005));
#7257=CARTESIAN_POINT('',(0.075,-0.045275768481829,-0.005));
#7258=CARTESIAN_POINT('Origin',(0.0775,-0.045275768481829,-0.005));
#7259=CARTESIAN_POINT('Origin',(0.0043,-0.045275768481829,-0.005));
#7260=CARTESIAN_POINT('',(0.0043,-0.058475768481829,0.));
#7261=CARTESIAN_POINT('',(0.0043,-0.032075768481829,0.));
#7262=CARTESIAN_POINT('',(0.0043,-0.045275768481829,0.));
#7263=CARTESIAN_POINT('',(0.0043,-0.058475768481829,-0.07));
#7264=CARTESIAN_POINT('',(0.0043,-0.058475768481829,-0.005));
#7265=CARTESIAN_POINT('',(0.0043,-0.032075768481829,-0.07));
#7266=CARTESIAN_POINT('',(0.0043,-0.045275768481829,-0.07));
#7267=CARTESIAN_POINT('',(0.0043,-0.032075768481829,-0.005));
#7268=CARTESIAN_POINT('Origin',(0.0175,-0.058475768481829,-0.005));
#7269=CARTESIAN_POINT('',(0.0307,-0.058475768481829,0.));
#7270=CARTESIAN_POINT('',(0.0175,-0.058475768481829,0.));
#7271=CARTESIAN_POINT('',(0.0307,-0.058475768481829,-0.07));
#7272=CARTESIAN_POINT('',(0.0307,-0.058475768481829,-0.005));
#7273=CARTESIAN_POINT('',(0.0175,-0.058475768481829,-0.07));
#7274=CARTESIAN_POINT('Origin',(0.0307,-0.045275768481829,-0.005));
#7275=CARTESIAN_POINT('',(0.0307,-0.032075768481829,0.));
#7276=CARTESIAN_POINT('',(0.0307,-0.045275768481829,0.));
#7277=CARTESIAN_POINT('',(0.0307,-0.032075768481829,-0.07));
#7278=CARTESIAN_POINT('',(0.0307,-0.032075768481829,-0.005));
#7279=CARTESIAN_POINT('',(0.0307,-0.045275768481829,-0.07));
#7280=CARTESIAN_POINT('',(0.0307,-0.045975768481829,-0.0375));
#7281=CARTESIAN_POINT('Origin',(0.0307,-0.045975768481829,-0.04));
#7282=CARTESIAN_POINT('Origin',(0.0475,-0.062775768481829,-0.005));
#7283=CARTESIAN_POINT('',(0.012,-0.062775768481829,0.));
#7284=CARTESIAN_POINT('',(0.012,-0.062775768481829,-0.068));
#7285=CARTESIAN_POINT('',(0.012,-0.062775768481829,-0.005));
#7286=CARTESIAN_POINT('',(0.095,-0.062775768481829,-0.068));
#7287=CARTESIAN_POINT('',(0.0475,-0.062775768481829,-0.068));
#7288=CARTESIAN_POINT('',(0.095,-0.062775768481829,0.));
#7289=CARTESIAN_POINT('',(0.095,-0.062775768481829,-0.005));
#7290=CARTESIAN_POINT('',(0.0475,-0.062775768481829,0.));
#7291=CARTESIAN_POINT('Origin',(0.,-0.015275768481829,-0.005));
#7292=CARTESIAN_POINT('',(-3.46944695195361E-18,0.032224231518171,-0.068));
#7293=CARTESIAN_POINT('',(-3.46944695195361E-18,0.032224231518171,0.));
#7294=CARTESIAN_POINT('',(-3.46944695195361E-18,0.032224231518171,-0.005));
#7295=CARTESIAN_POINT('',(0.,-0.050775768481829,-0.068));
#7296=CARTESIAN_POINT('',(0.,-0.015275768481829,-0.068));
#7297=CARTESIAN_POINT('',(0.,-0.050775768481829,0.));
#7298=CARTESIAN_POINT('',(0.,-0.050775768481829,-0.005));
#7299=CARTESIAN_POINT('',(0.,-0.015275768481829,0.));
#7300=CARTESIAN_POINT('Origin',(0.0175,0.032224231518171,-0.005));
#7301=CARTESIAN_POINT('',(0.012,0.032224231518171,-0.08));
#7302=CARTESIAN_POINT('',(0.035,0.032224231518171,-0.08));
#7303=CARTESIAN_POINT('',(0.0175,0.032224231518171,-0.08));
#7304=CARTESIAN_POINT('Origin',(0.012,0.032224231518171,-0.068));
#7305=CARTESIAN_POINT('',(0.035,0.032224231518171,0.));
#7306=CARTESIAN_POINT('',(0.0175,0.032224231518171,0.));
#7307=CARTESIAN_POINT('',(0.035,0.032224231518171,-0.005));
#7308=CARTESIAN_POINT('',(0.035,0.032224231518171,-0.005));
#7309=CARTESIAN_POINT('',(0.0043,0.032224231518171,-0.005));
#7310=CARTESIAN_POINT('',(0.0175,0.032224231518171,-0.005));
#7311=CARTESIAN_POINT('',(0.0043,0.032224231518171,-0.07));
#7312=CARTESIAN_POINT('',(0.0043,0.032224231518171,-0.07));
#7313=CARTESIAN_POINT('',(0.035,0.032224231518171,-0.07));
#7314=CARTESIAN_POINT('',(0.0175,0.032224231518171,-0.07));
#7315=CARTESIAN_POINT('',(0.035,0.032224231518171,-0.08));
#7316=CARTESIAN_POINT('Origin',(0.035,0.002224231518171,-0.005));
#7317=CARTESIAN_POINT('',(0.035,-0.027775768481829,0.));
#7318=CARTESIAN_POINT('',(0.035,0.002224231518171,0.));
#7319=CARTESIAN_POINT('',(0.035,-0.027775768481829,-0.005));
#7320=CARTESIAN_POINT('',(0.035,0.002224231518171,-0.005));
#7321=CARTESIAN_POINT('Origin',(0.065,-0.027775768481829,-0.005));
#7322=CARTESIAN_POINT('',(0.095,-0.027775768481829,0.));
#7323=CARTESIAN_POINT('',(0.065,-0.027775768481829,0.));
#7324=CARTESIAN_POINT('',(0.095,-0.027775768481829,-0.005));
#7325=CARTESIAN_POINT('Origin',(0.0175,0.014724231518171,-0.005));
#7326=CARTESIAN_POINT('',(0.015,0.014724231518171,-0.005));
#7327=CARTESIAN_POINT('Origin',(0.0175,0.014724231518171,-0.005));
#7328=CARTESIAN_POINT('',(0.015,0.014724231518171,0.));
#7329=CARTESIAN_POINT('',(0.015,0.014724231518171,-0.005));
#7330=CARTESIAN_POINT('Origin',(0.0175,0.014724231518171,0.));
#7331=CARTESIAN_POINT('Origin',(0.0175,-0.032075768481829,-0.005));
#7332=CARTESIAN_POINT('',(0.0175,-0.032075768481829,0.));
#7333=CARTESIAN_POINT('',(0.0175,-0.032075768481829,-0.07));
#7334=CARTESIAN_POINT('',(0.0168,-0.032075768481829,-0.0425));
#7335=CARTESIAN_POINT('Origin',(0.0168,-0.032075768481829,-0.04));
#7336=CARTESIAN_POINT('Origin',(0.095,-0.045275768481829,-0.005));
#7337=CARTESIAN_POINT('',(0.095,-0.050775768481829,-0.08));
#7338=CARTESIAN_POINT('Origin',(0.095,-0.050775768481829,-0.068));
#7339=CARTESIAN_POINT('',(0.095,-0.027775768481829,-0.08));
#7340=CARTESIAN_POINT('',(0.095,-0.045275768481829,-0.08));
#7341=CARTESIAN_POINT('',(0.095,-0.027775768481829,-0.07));
#7342=CARTESIAN_POINT('',(0.095,-0.027775768481829,-0.08));
#7343=CARTESIAN_POINT('',(0.095,-0.058475768481829,-0.07));
#7344=CARTESIAN_POINT('',(0.095,-0.045275768481829,-0.07));
#7345=CARTESIAN_POINT('',(0.095,-0.058475768481829,-0.07));
#7346=CARTESIAN_POINT('',(0.095,-0.045275768481829,0.));
#7347=CARTESIAN_POINT('Origin',(0.0775,-0.045275768481829,-0.005));
#7348=CARTESIAN_POINT('',(0.075,-0.045275768481829,0.));
#7349=CARTESIAN_POINT('',(0.075,-0.045275768481829,-0.005));
#7350=CARTESIAN_POINT('Origin',(0.0775,-0.045275768481829,0.));
#7351=CARTESIAN_POINT('Origin',(0.0475,-0.015275768481829,-0.005));
#7352=CARTESIAN_POINT('',(0.0043,-0.027775768481829,-0.005));
#7353=CARTESIAN_POINT('',(0.0043,0.002224231518171,-0.005));
#7354=CARTESIAN_POINT('',(0.01965,-0.027775768481829,-0.005));
#7355=CARTESIAN_POINT('Origin',(0.0475,-0.015275768481829,0.));
#7356=CARTESIAN_POINT('Origin',(0.012,-0.050775768481829,0.));
#7357=CARTESIAN_POINT('Origin',(0.035,-0.043125768481829,-0.07));
#7358=CARTESIAN_POINT('',(0.035,-0.058475768481829,-0.07));
#7359=CARTESIAN_POINT('',(0.035,-0.058475768481829,-0.07));
#7360=CARTESIAN_POINT('',(0.035,-0.027775768481829,-0.07));
#7361=CARTESIAN_POINT('',(0.035,-0.043125768481829,-0.07));
#7362=CARTESIAN_POINT('',(0.035,-0.027775768481829,-0.07));
#7363=CARTESIAN_POINT('',(0.035,-0.045975768481829,-0.0375));
#7364=CARTESIAN_POINT('Origin',(0.035,-0.045975768481829,-0.04));
#7365=CARTESIAN_POINT('Origin',(0.065,-0.058475768481829,-0.07));
#7366=CARTESIAN_POINT('',(0.065,-0.058475768481829,-0.07));
#7367=CARTESIAN_POINT('Origin',(0.0043,0.002224231518171,-0.07));
#7368=CARTESIAN_POINT('',(0.0043,-0.027775768481829,-0.07));
#7369=CARTESIAN_POINT('',(0.0043,-0.027775768481829,-0.07));
#7370=CARTESIAN_POINT('',(0.0043,0.002224231518171,-0.07));
#7371=CARTESIAN_POINT('Origin',(0.01965,-0.027775768481829,-0.07));
#7372=CARTESIAN_POINT('',(0.01965,-0.027775768481829,-0.07));
#7373=CARTESIAN_POINT('',(0.0168,-0.027775768481829,-0.0425));
#7374=CARTESIAN_POINT('Origin',(0.0168,-0.027775768481829,-0.04));
#7375=CARTESIAN_POINT('Origin',(0.025,-0.045975768481829,-0.04));
#7376=CARTESIAN_POINT('',(0.025,-0.045975768481829,-0.0375));
#7377=CARTESIAN_POINT('Origin',(0.0168,-0.037775768481829,-0.04));
#7378=CARTESIAN_POINT('',(0.0168,-0.037775768481829,-0.0425));
#7379=CARTESIAN_POINT('Origin',(0.0475,-0.015275768481829,-0.08));
#7380=CARTESIAN_POINT('',(0.012,-0.050775768481829,-0.08));
#7381=CARTESIAN_POINT('',(0.0475,-0.050775768481829,-0.08));
#7382=CARTESIAN_POINT('',(0.012,-0.015275768481829,-0.08));
#7383=CARTESIAN_POINT('',(0.035,-0.027775768481829,-0.08));
#7384=CARTESIAN_POINT('',(0.035,0.002224231518171,-0.08));
#7385=CARTESIAN_POINT('',(0.065,-0.027775768481829,-0.08));
#7386=CARTESIAN_POINT('Origin',(0.065,-0.027775768481829,-0.08));
#7387=CARTESIAN_POINT('',(0.065,-0.027775768481829,-0.07));
#7388=CARTESIAN_POINT('',(0.035,-0.027775768481829,-0.08));
#7389=CARTESIAN_POINT('Origin',(0.035,0.002224231518171,-0.08));
#7390=CARTESIAN_POINT('',(0.035,0.002224231518171,-0.07));
#7391=CARTESIAN_POINT('Origin',(0.0475,-0.015275768481829,-0.07));
#7392=CARTESIAN_POINT('Origin',(0.0475,-0.015275768481829,-0.07));
#7393=CARTESIAN_POINT('Origin',(0.0475,-0.015275768481829,-0.07));
#7394=CARTESIAN_POINT('Origin',(0.012,-0.050775768481829,-0.005));
#7395=CARTESIAN_POINT('Origin',(0.012,-0.050775768481829,-0.068));
#7396=CARTESIAN_POINT('Origin',(0.012,-0.015275768481829,-0.068));
#7397=CARTESIAN_POINT('Origin',(0.012,-0.050775768481829,-0.068));
#7398=CARTESIAN_POINT('Origin',(0.0475,-0.050775768481829,-0.068));
#7399=CARTESIAN_POINT('Origin',(0.012,-0.050775768481829,-0.068));
#7400=CARTESIAN_POINT('Origin',(0.012,-0.050775768481829,-0.068));
#7743=UNCERTAINTY_MEASURE_WITH_UNIT(LENGTH_MEASURE(1.E-5),#7757,
'DISTANCE_ACCURACY_VALUE',
'Maximum model space distance between geometric entities at asserted c
onnectivities');
#7745=UNCERTAINTY_MEASURE_WITH_UNIT(LENGTH_MEASURE(1.E-5),#7757,
'DISTANCE_ACCURACY_VALUE',
'Maximum model space distance between geometric entities at asserted c
onnectivities');
#7754=(
GEOMETRIC_REPRESENTATION_CONTEXT(3)
GLOBAL_UNCERTAINTY_ASSIGNED_CONTEXT((#7743))
GLOBAL_UNIT_ASSIGNED_CONTEXT((#7757,#7758,#7759))
REPRESENTATION_CONTEXT('','3D')
);
#7756=(
GEOMETRIC_REPRESENTATION_CONTEXT(3)
GLOBAL_UNCERTAINTY_ASSIGNED_CONTEXT((#7745))
GLOBAL_UNIT_ASSIGNED_CONTEXT((#7757,#7758,#7759))
REPRESENTATION_CONTEXT('','3D')
);
#7757=(
LENGTH_UNIT()
NAMED_UNIT(*)
SI_UNIT($,.METRE.)
);
#7758=(
NAMED_UNIT(*)
PLANE_ANGLE_UNIT()
SI_UNIT($,.RADIAN.)
);
#7759=(
NAMED_UNIT(*)
SI_UNIT($,.STERADIAN.)
SOLID_ANGLE_UNIT()
);
#7768=SHAPE_DEFINITION_REPRESENTATION(#7778,#7826);
#7778=PRODUCT_DEFINITION_SHAPE('',$,#7837);
#7826=SHAPE_REPRESENTATION('',(#4957),#7754);
#7828=PRODUCT_DEFINITION_CONTEXT('part definition',#7860,'design');
#7837=PRODUCT_DEFINITION('Corner Electronics Bay Bracket',
'Corner Electronics Bay Bracket',#7847,#7828);
#7847=PRODUCT_DEFINITION_FORMATION('',$,#7870);
#7860=APPLICATION_CONTEXT(
'Core Data for Automotive Mechanical Design Process');
#7861=PRODUCT_CONTEXT('part definition',#7860,'mechanical');
#7870=PRODUCT('Corner Electronics Bay Bracket',
'Corner Electronics Bay Bracket',
'LEGAL AND USAGE DISCLAIMER: this Data/Model is provided \X2\201C\X0\A
S IS\X2\201D\X0\ for informational and representational only. It is a 
geometric approximation and is NOT engineered, certified, or guarantee
d for dimensional accuracy, exact tolerances, or production-level prec
ision. Vendor disclaims all implied warranties including fitness for a
 particular purpose. DO NOT USE FOR DIRECT PHYSICAL MANUFACTURING, AUT
OMATED PRODUCTION, OR SAFETY-CRITICAL SYSTEMS without independent engi
neering verification and resolution of any design discrepancies.',(#7861));
#7874=PRESENTATION_STYLE_ASSIGNMENT((#7881));
#7881=SURFACE_STYLE_USAGE(.BOTH.,#7888);
#7888=SURFACE_SIDE_STYLE('',(#7895));
#7895=SURFACE_STYLE_FILL_AREA(#7902);
#7902=FILL_AREA_STYLE('Opaque(179,179,179)',(#7909));
#7909=FILL_AREA_STYLE_COLOUR('Opaque(179,179,179)',#7916);
#7916=COLOUR_RGB('Opaque(179,179,179)',0.701960784313725,0.701960784313725,
0.701960784313725);
ENDSEC;
END-ISO-10303-21;
